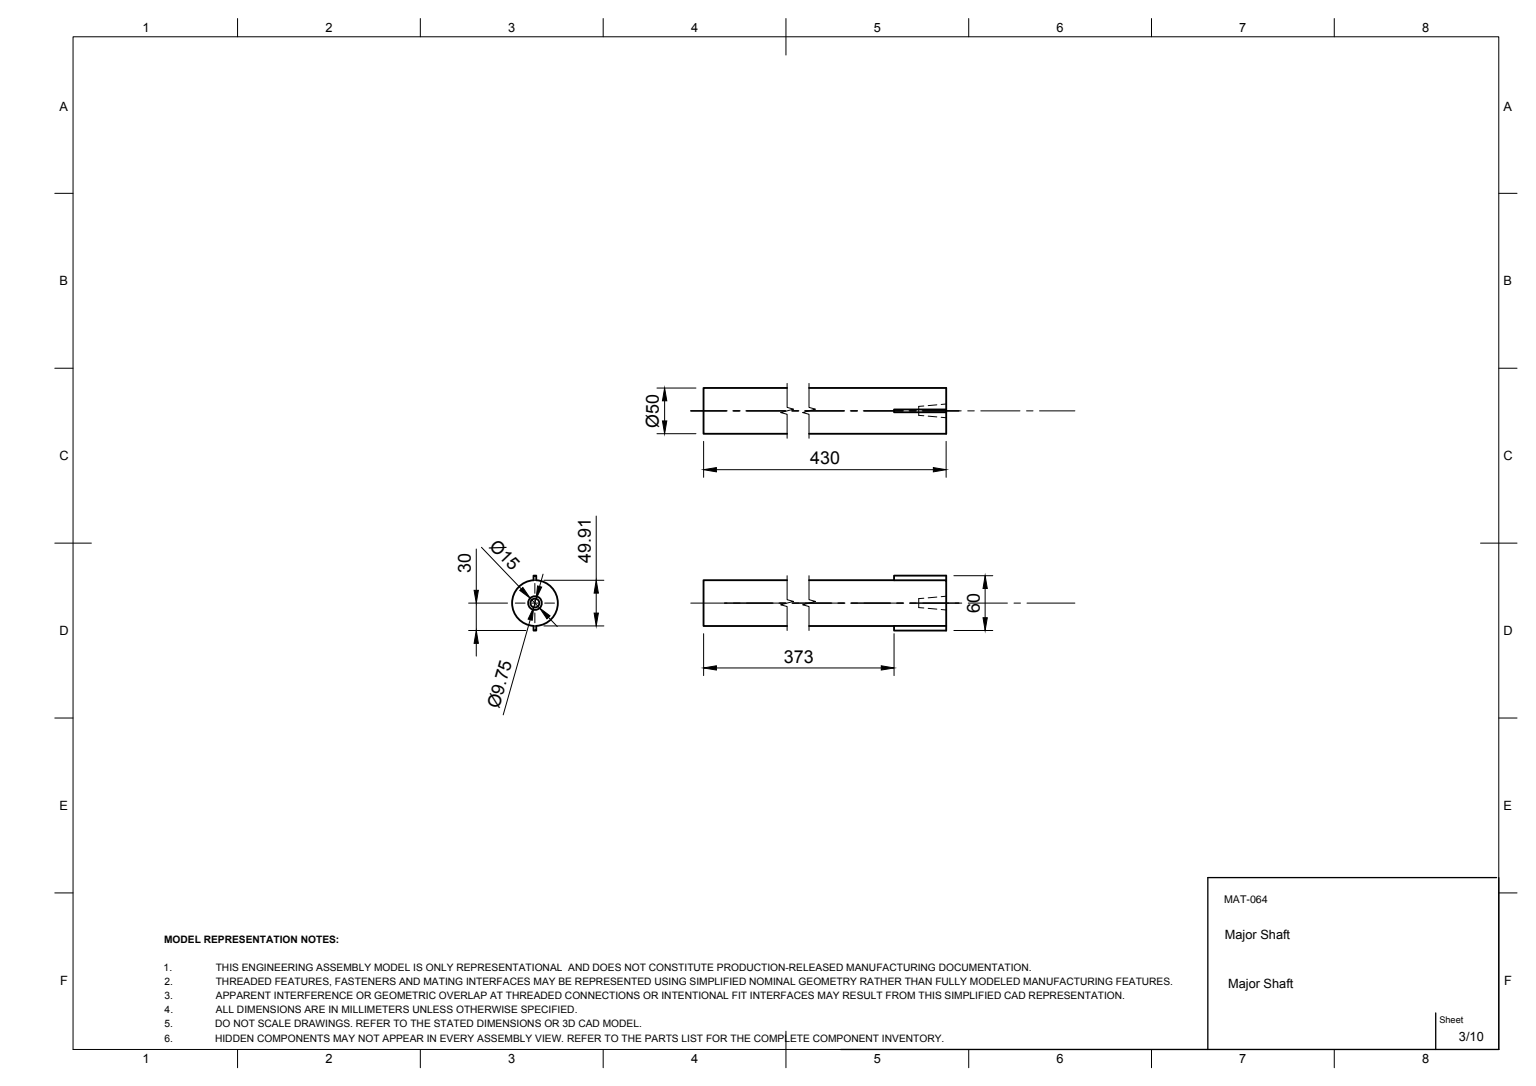
ISO-10303-21;
HEADER;
/* Generated by software containing ST-Developer
 * from STEP Tools, Inc. (www.steptools.com) 
 */

FILE_DESCRIPTION(
/* description */ (''),
/* implementation_level */ '2;1');

FILE_NAME(
/* name */ 
'Major Shaft.step',
/* time_stamp */ '2026-10-24T12:42:14-07:00',
/* author */ (''),
/* organization */ (''),
/* preprocessor_version */ 'ST-DEVELOPER v20.2',
/* originating_system */ 'Autodesk Translation Framework v15.15.0.0',
/* authorisation */ '');

FILE_SCHEMA (('AUTOMOTIVE_DESIGN { 1 0 10303 214 3 1 1 }'));
ENDSEC;

DATA;
#10=MECHANICAL_DESIGN_GEOMETRIC_PRESENTATION_REPRESENTATION('',(#68),#6789);
#15=CONICAL_SURFACE('',#4306,7.5,0.0872664625997165);
#56=SHAPE_REPRESENTATION_RELATIONSHIP('SRR','None',#6823,#62);
#62=ADVANCED_BREP_SHAPE_REPRESENTATION('',(#74),#6785);
#68=STYLED_ITEM('',(#6863),#74);
#74=MANIFOLD_SOLID_BREP('Major Shaft',#3963);
#160=CYLINDRICAL_SURFACE('',#4288,25.);
#219=FACE_BOUND('',#797,.T.);
#322=CIRCLE('',#4289,25.);
#323=CIRCLE('',#4290,25.);
#324=CIRCLE('',#4291,25.);
#325=CIRCLE('',#4292,25.);
#326=CIRCLE('',#4293,25.);
#327=CIRCLE('',#4294,25.);
#328=CIRCLE('',#4296,7.5);
#329=CIRCLE('',#4307,4.87534009422228);
#544=FACE_OUTER_BOUND('',#795,.T.);
#545=FACE_OUTER_BOUND('',#796,.T.);
#546=FACE_OUTER_BOUND('',#798,.T.);
#547=FACE_OUTER_BOUND('',#799,.T.);
#548=FACE_OUTER_BOUND('',#800,.T.);
#549=FACE_OUTER_BOUND('',#801,.T.);
#550=FACE_OUTER_BOUND('',#802,.T.);
#551=FACE_OUTER_BOUND('',#803,.T.);
#552=FACE_OUTER_BOUND('',#804,.T.);
#553=FACE_OUTER_BOUND('',#805,.T.);
#554=FACE_OUTER_BOUND('',#806,.T.);
#555=FACE_OUTER_BOUND('',#807,.T.);
#556=FACE_OUTER_BOUND('',#808,.T.);
#795=EDGE_LOOP('',(#3345,#3346,#3347,#3348,#3349,#3350,#3351,#3352,#3353,
#3354,#3355,#3356));
#796=EDGE_LOOP('',(#3357,#3358,#3359,#3360,#3361,#3362,#3363,#3364));
#797=EDGE_LOOP('',(#3365));
#798=EDGE_LOOP('',(#3366));
#799=EDGE_LOOP('',(#3367,#3368,#3369,#3370,#3371));
#800=EDGE_LOOP('',(#3372,#3373,#3374,#3375));
#801=EDGE_LOOP('',(#3376,#3377,#3378,#3379));
#802=EDGE_LOOP('',(#3380,#3381,#3382,#3383));
#803=EDGE_LOOP('',(#3384,#3385,#3386,#3387));
#804=EDGE_LOOP('',(#3388,#3389,#3390,#3391));
#805=EDGE_LOOP('',(#3392,#3393,#3394,#3395));
#806=EDGE_LOOP('',(#3396,#3397,#3398,#3399));
#807=EDGE_LOOP('',(#3400,#3401,#3402,#3403));
#808=EDGE_LOOP('',(#3404));
#1195=LINE('',#6434,#1573);
#1196=LINE('',#6438,#1574);
#1197=LINE('',#6442,#1575);
#1198=LINE('',#6446,#1576);
#1199=LINE('',#6450,#1577);
#1200=LINE('',#6454,#1578);
#1201=LINE('',#6456,#1579);
#1202=LINE('',#6457,#1580);
#1203=LINE('',#6459,#1581);
#1204=LINE('',#6461,#1582);
#1205=LINE('',#6462,#1583);
#1206=LINE('',#6469,#1584);
#1207=LINE('',#6470,#1585);
#1208=LINE('',#6471,#1586);
#1209=LINE('',#6473,#1587);
#1210=LINE('',#6475,#1588);
#1211=LINE('',#6479,#1589);
#1212=LINE('',#6481,#1590);
#1213=LINE('',#6482,#1591);
#1214=LINE('',#6484,#1592);
#1215=LINE('',#6486,#1593);
#1216=LINE('',#6491,#1594);
#1573=VECTOR('',#5254,25.);
#1574=VECTOR('',#5257,57.0000000000001);
#1575=VECTOR('',#5260,57.0000000000001);
#1576=VECTOR('',#5263,57.0000000000001);
#1577=VECTOR('',#5266,57.0000000000001);
#1578=VECTOR('',#5271,5.04504057306444);
#1579=VECTOR('',#5272,3.);
#1580=VECTOR('',#5273,5.04504057306444);
#1581=VECTOR('',#5274,5.04504057306444);
#1582=VECTOR('',#5275,3.);
#1583=VECTOR('',#5276,5.04504057306444);
#1584=VECTOR('',#5283,3.);
#1585=VECTOR('',#5284,5.04504057306444);
#1586=VECTOR('',#5285,5.04504057306444);
#1587=VECTOR('',#5288,57.0000000000001);
#1588=VECTOR('',#5291,57.0000000000001);
#1589=VECTOR('',#5296,5.04504057306444);
#1590=VECTOR('',#5297,3.);
#1591=VECTOR('',#5298,5.04504057306444);
#1592=VECTOR('',#5301,57.0000000000001);
#1593=VECTOR('',#5304,57.0000000000001);
#1594=VECTOR('',#5311,7.5);
#1901=VERTEX_POINT('',#6431);
#1902=VERTEX_POINT('',#6433);
#1903=VERTEX_POINT('',#6435);
#1904=VERTEX_POINT('',#6437);
#1905=VERTEX_POINT('',#6439);
#1906=VERTEX_POINT('',#6441);
#1907=VERTEX_POINT('',#6443);
#1908=VERTEX_POINT('',#6445);
#1909=VERTEX_POINT('',#6447);
#1910=VERTEX_POINT('',#6449);
#1911=VERTEX_POINT('',#6453);
#1912=VERTEX_POINT('',#6455);
#1913=VERTEX_POINT('',#6458);
#1914=VERTEX_POINT('',#6460);
#1915=VERTEX_POINT('',#6463);
#1916=VERTEX_POINT('',#6467);
#1917=VERTEX_POINT('',#6468);
#1918=VERTEX_POINT('',#6478);
#1919=VERTEX_POINT('',#6480);
#1920=VERTEX_POINT('',#6489);
#2393=EDGE_CURVE('',#1901,#1901,#322,.T.);
#2394=EDGE_CURVE('',#1901,#1902,#1195,.T.);
#2395=EDGE_CURVE('',#1902,#1903,#323,.T.);
#2396=EDGE_CURVE('',#1903,#1904,#1196,.T.);
#2397=EDGE_CURVE('',#1904,#1905,#324,.T.);
#2398=EDGE_CURVE('',#1906,#1905,#1197,.T.);
#2399=EDGE_CURVE('',#1906,#1907,#325,.T.);
#2400=EDGE_CURVE('',#1907,#1908,#1198,.T.);
#2401=EDGE_CURVE('',#1908,#1909,#326,.T.);
#2402=EDGE_CURVE('',#1910,#1909,#1199,.T.);
#2403=EDGE_CURVE('',#1910,#1902,#327,.T.);
#2404=EDGE_CURVE('',#1908,#1911,#1200,.T.);
#2405=EDGE_CURVE('',#1911,#1912,#1201,.T.);
#2406=EDGE_CURVE('',#1912,#1905,#1202,.T.);
#2407=EDGE_CURVE('',#1904,#1913,#1203,.T.);
#2408=EDGE_CURVE('',#1913,#1914,#1204,.T.);
#2409=EDGE_CURVE('',#1914,#1909,#1205,.T.);
#2410=EDGE_CURVE('',#1915,#1915,#328,.T.);
#2411=EDGE_CURVE('',#1916,#1917,#1206,.T.);
#2412=EDGE_CURVE('',#1903,#1916,#1207,.T.);
#2413=EDGE_CURVE('',#1917,#1910,#1208,.T.);
#2414=EDGE_CURVE('',#1917,#1914,#1209,.T.);
#2415=EDGE_CURVE('',#1916,#1913,#1210,.T.);
#2416=EDGE_CURVE('',#1918,#1906,#1211,.T.);
#2417=EDGE_CURVE('',#1919,#1918,#1212,.T.);
#2418=EDGE_CURVE('',#1907,#1919,#1213,.T.);
#2419=EDGE_CURVE('',#1919,#1911,#1214,.T.);
#2420=EDGE_CURVE('',#1918,#1912,#1215,.T.);
#2421=EDGE_CURVE('',#1920,#1920,#329,.T.);
#2422=EDGE_CURVE('',#1920,#1915,#1216,.T.);
#3345=ORIENTED_EDGE('',*,*,#2393,.F.);
#3346=ORIENTED_EDGE('',*,*,#2394,.T.);
#3347=ORIENTED_EDGE('',*,*,#2395,.T.);
#3348=ORIENTED_EDGE('',*,*,#2396,.T.);
#3349=ORIENTED_EDGE('',*,*,#2397,.T.);
#3350=ORIENTED_EDGE('',*,*,#2398,.F.);
#3351=ORIENTED_EDGE('',*,*,#2399,.T.);
#3352=ORIENTED_EDGE('',*,*,#2400,.T.);
#3353=ORIENTED_EDGE('',*,*,#2401,.T.);
#3354=ORIENTED_EDGE('',*,*,#2402,.F.);
#3355=ORIENTED_EDGE('',*,*,#2403,.T.);
#3356=ORIENTED_EDGE('',*,*,#2394,.F.);
#3357=ORIENTED_EDGE('',*,*,#2401,.F.);
#3358=ORIENTED_EDGE('',*,*,#2404,.T.);
#3359=ORIENTED_EDGE('',*,*,#2405,.T.);
#3360=ORIENTED_EDGE('',*,*,#2406,.T.);
#3361=ORIENTED_EDGE('',*,*,#2397,.F.);
#3362=ORIENTED_EDGE('',*,*,#2407,.T.);
#3363=ORIENTED_EDGE('',*,*,#2408,.T.);
#3364=ORIENTED_EDGE('',*,*,#2409,.T.);
#3365=ORIENTED_EDGE('',*,*,#2410,.F.);
#3366=ORIENTED_EDGE('',*,*,#2393,.T.);
#3367=ORIENTED_EDGE('',*,*,#2411,.F.);
#3368=ORIENTED_EDGE('',*,*,#2412,.F.);
#3369=ORIENTED_EDGE('',*,*,#2395,.F.);
#3370=ORIENTED_EDGE('',*,*,#2403,.F.);
#3371=ORIENTED_EDGE('',*,*,#2413,.F.);
#3372=ORIENTED_EDGE('',*,*,#2414,.F.);
#3373=ORIENTED_EDGE('',*,*,#2413,.T.);
#3374=ORIENTED_EDGE('',*,*,#2402,.T.);
#3375=ORIENTED_EDGE('',*,*,#2409,.F.);
#3376=ORIENTED_EDGE('',*,*,#2396,.F.);
#3377=ORIENTED_EDGE('',*,*,#2412,.T.);
#3378=ORIENTED_EDGE('',*,*,#2415,.T.);
#3379=ORIENTED_EDGE('',*,*,#2407,.F.);
#3380=ORIENTED_EDGE('',*,*,#2415,.F.);
#3381=ORIENTED_EDGE('',*,*,#2411,.T.);
#3382=ORIENTED_EDGE('',*,*,#2414,.T.);
#3383=ORIENTED_EDGE('',*,*,#2408,.F.);
#3384=ORIENTED_EDGE('',*,*,#2416,.F.);
#3385=ORIENTED_EDGE('',*,*,#2417,.F.);
#3386=ORIENTED_EDGE('',*,*,#2418,.F.);
#3387=ORIENTED_EDGE('',*,*,#2399,.F.);
#3388=ORIENTED_EDGE('',*,*,#2400,.F.);
#3389=ORIENTED_EDGE('',*,*,#2418,.T.);
#3390=ORIENTED_EDGE('',*,*,#2419,.T.);
#3391=ORIENTED_EDGE('',*,*,#2404,.F.);
#3392=ORIENTED_EDGE('',*,*,#2419,.F.);
#3393=ORIENTED_EDGE('',*,*,#2417,.T.);
#3394=ORIENTED_EDGE('',*,*,#2420,.T.);
#3395=ORIENTED_EDGE('',*,*,#2405,.F.);
#3396=ORIENTED_EDGE('',*,*,#2420,.F.);
#3397=ORIENTED_EDGE('',*,*,#2416,.T.);
#3398=ORIENTED_EDGE('',*,*,#2398,.T.);
#3399=ORIENTED_EDGE('',*,*,#2406,.F.);
#3400=ORIENTED_EDGE('',*,*,#2421,.F.);
#3401=ORIENTED_EDGE('',*,*,#2422,.T.);
#3402=ORIENTED_EDGE('',*,*,#2410,.T.);
#3403=ORIENTED_EDGE('',*,*,#2422,.F.);
#3404=ORIENTED_EDGE('',*,*,#2421,.T.);
#3715=PLANE('',#4295);
#3716=PLANE('',#4297);
#3717=PLANE('',#4298);
#3718=PLANE('',#4299);
#3719=PLANE('',#4300);
#3720=PLANE('',#4301);
#3721=PLANE('',#4302);
#3722=PLANE('',#4303);
#3723=PLANE('',#4304);
#3724=PLANE('',#4305);
#3725=PLANE('',#4308);
#3894=ADVANCED_FACE('',(#544),#160,.T.);
#3895=ADVANCED_FACE('',(#545,#219),#3715,.F.);
#3896=ADVANCED_FACE('',(#546),#3716,.T.);
#3897=ADVANCED_FACE('',(#547),#3717,.T.);
#3898=ADVANCED_FACE('',(#548),#3718,.T.);
#3899=ADVANCED_FACE('',(#549),#3719,.T.);
#3900=ADVANCED_FACE('',(#550),#3720,.T.);
#3901=ADVANCED_FACE('',(#551),#3721,.T.);
#3902=ADVANCED_FACE('',(#552),#3722,.T.);
#3903=ADVANCED_FACE('',(#553),#3723,.T.);
#3904=ADVANCED_FACE('',(#554),#3724,.T.);
#3905=ADVANCED_FACE('',(#555),#15,.F.);
#3906=ADVANCED_FACE('',(#556),#3725,.T.);
#3963=CLOSED_SHELL('',(#3894,#3895,#3896,#3897,#3898,#3899,#3900,#3901,
#3902,#3903,#3904,#3905,#3906));
#4287=AXIS2_PLACEMENT_3D('',#6429,#5248,#5249);
#4288=AXIS2_PLACEMENT_3D('',#6430,#5250,#5251);
#4289=AXIS2_PLACEMENT_3D('',#6432,#5252,#5253);
#4290=AXIS2_PLACEMENT_3D('',#6436,#5255,#5256);
#4291=AXIS2_PLACEMENT_3D('',#6440,#5258,#5259);
#4292=AXIS2_PLACEMENT_3D('',#6444,#5261,#5262);
#4293=AXIS2_PLACEMENT_3D('',#6448,#5264,#5265);
#4294=AXIS2_PLACEMENT_3D('',#6451,#5267,#5268);
#4295=AXIS2_PLACEMENT_3D('',#6452,#5269,#5270);
#4296=AXIS2_PLACEMENT_3D('',#6464,#5277,#5278);
#4297=AXIS2_PLACEMENT_3D('',#6465,#5279,#5280);
#4298=AXIS2_PLACEMENT_3D('',#6466,#5281,#5282);
#4299=AXIS2_PLACEMENT_3D('',#6472,#5286,#5287);
#4300=AXIS2_PLACEMENT_3D('',#6474,#5289,#5290);
#4301=AXIS2_PLACEMENT_3D('',#6476,#5292,#5293);
#4302=AXIS2_PLACEMENT_3D('',#6477,#5294,#5295);
#4303=AXIS2_PLACEMENT_3D('',#6483,#5299,#5300);
#4304=AXIS2_PLACEMENT_3D('',#6485,#5302,#5303);
#4305=AXIS2_PLACEMENT_3D('',#6487,#5305,#5306);
#4306=AXIS2_PLACEMENT_3D('',#6488,#5307,#5308);
#4307=AXIS2_PLACEMENT_3D('',#6490,#5309,#5310);
#4308=AXIS2_PLACEMENT_3D('',#6492,#5312,#5313);
#5248=DIRECTION('axis',(0.,0.,1.));
#5249=DIRECTION('refdir',(1.,0.,0.));
#5250=DIRECTION('center_axis',(0.,-1.,0.));
#5251=DIRECTION('ref_axis',(0.,0.,-1.));
#5252=DIRECTION('center_axis',(0.,-1.,0.));
#5253=DIRECTION('ref_axis',(0.,0.,-1.));
#5254=DIRECTION('',(0.,1.,0.));
#5255=DIRECTION('center_axis',(0.,-1.,0.));
#5256=DIRECTION('ref_axis',(0.,0.,-1.));
#5257=DIRECTION('',(0.,1.,0.));
#5258=DIRECTION('center_axis',(0.,-1.,0.));
#5259=DIRECTION('ref_axis',(0.,0.,-1.));
#5260=DIRECTION('',(0.,1.,0.));
#5261=DIRECTION('center_axis',(0.,-1.,0.));
#5262=DIRECTION('ref_axis',(0.,0.,-1.));
#5263=DIRECTION('',(0.,1.,0.));
#5264=DIRECTION('center_axis',(0.,-1.,0.));
#5265=DIRECTION('ref_axis',(0.,0.,-1.));
#5266=DIRECTION('',(0.,1.,0.));
#5267=DIRECTION('center_axis',(0.,-1.,0.));
#5268=DIRECTION('ref_axis',(0.,0.,-1.));
#5269=DIRECTION('center_axis',(0.,-1.,0.));
#5270=DIRECTION('ref_axis',(0.,0.,-1.));
#5271=DIRECTION('',(2.75077823593892E-16,0.,-1.));
#5272=DIRECTION('',(-1.,0.,0.));
#5273=DIRECTION('',(4.95140082469005E-16,0.,1.));
#5274=DIRECTION('',(-4.95140082469005E-16,0.,1.));
#5275=DIRECTION('',(1.,0.,0.));
#5276=DIRECTION('',(-2.75077823593892E-16,0.,-1.));
#5277=DIRECTION('center_axis',(0.,1.,0.));
#5278=DIRECTION('ref_axis',(0.,0.,1.));
#5279=DIRECTION('center_axis',(0.,-1.,0.));
#5280=DIRECTION('ref_axis',(0.,0.,-1.));
#5281=DIRECTION('center_axis',(0.,-1.,0.));
#5282=DIRECTION('ref_axis',(0.,0.,-1.));
#5283=DIRECTION('',(1.,0.,0.));
#5284=DIRECTION('',(-4.95140082469005E-16,0.,1.));
#5285=DIRECTION('',(-2.75077823593892E-16,0.,-1.));
#5286=DIRECTION('center_axis',(1.,0.,-3.00866369555819E-16));
#5287=DIRECTION('ref_axis',(-3.00866369555819E-16,0.,-1.));
#5288=DIRECTION('',(0.,1.,0.));
#5289=DIRECTION('center_axis',(-1.,0.,-4.72790009302002E-16));
#5290=DIRECTION('ref_axis',(-4.72790009302002E-16,0.,1.));
#5291=DIRECTION('',(0.,1.,0.));
#5292=DIRECTION('center_axis',(0.,0.,1.));
#5293=DIRECTION('ref_axis',(1.,0.,0.));
#5294=DIRECTION('center_axis',(0.,-1.,0.));
#5295=DIRECTION('ref_axis',(0.,0.,-1.));
#5296=DIRECTION('',(4.95140082469005E-16,0.,1.));
#5297=DIRECTION('',(-1.,0.,0.));
#5298=DIRECTION('',(2.75077823593892E-16,0.,-1.));
#5299=DIRECTION('center_axis',(1.,0.,3.00866369555819E-16));
#5300=DIRECTION('ref_axis',(3.00866369555819E-16,0.,-1.));
#5301=DIRECTION('',(0.,1.,0.));
#5302=DIRECTION('center_axis',(0.,0.,-1.));
#5303=DIRECTION('ref_axis',(-1.,0.,0.));
#5304=DIRECTION('',(0.,1.,0.));
#5305=DIRECTION('center_axis',(-1.,0.,4.72790009302002E-16));
#5306=DIRECTION('ref_axis',(4.72790009302002E-16,0.,1.));
#5307=DIRECTION('center_axis',(0.,1.,0.));
#5308=DIRECTION('ref_axis',(0.,0.,1.));
#5309=DIRECTION('center_axis',(0.,1.,0.));
#5310=DIRECTION('ref_axis',(0.,0.,1.));
#5311=DIRECTION('',(-1.0673500138323E-17,0.996194698091745,-0.0871557427476582));
#5312=DIRECTION('center_axis',(0.,1.,0.));
#5313=DIRECTION('ref_axis',(0.,0.,1.));
#6429=CARTESIAN_POINT('',(0.,0.,0.));
#6430=CARTESIAN_POINT('Origin',(0.,42.0000000000001,0.));
#6431=CARTESIAN_POINT('',(-3.06161699786838E-15,-388.,25.));
#6432=CARTESIAN_POINT('Origin',(0.,-388.,0.));
#6433=CARTESIAN_POINT('',(-3.06161699786838E-15,-15.,25.));
#6434=CARTESIAN_POINT('',(-3.06161699786838E-15,42.0000000000001,25.));
#6435=CARTESIAN_POINT('',(-1.5,-15.,24.9549594269356));
#6436=CARTESIAN_POINT('Origin',(0.,-15.,0.));
#6437=CARTESIAN_POINT('',(-1.5,42.0000000000001,24.9549594269356));
#6438=CARTESIAN_POINT('',(-1.5,-15.,24.9549594269356));
#6439=CARTESIAN_POINT('',(-1.5,42.0000000000001,-24.9549594269356));
#6440=CARTESIAN_POINT('Origin',(0.,42.0000000000001,0.));
#6441=CARTESIAN_POINT('',(-1.5,-15.,-24.9549594269356));
#6442=CARTESIAN_POINT('',(-1.49999999999999,-15.,-24.9549594269356));
#6443=CARTESIAN_POINT('',(1.5,-15.,-24.9549594269356));
#6444=CARTESIAN_POINT('Origin',(0.,-15.,0.));
#6445=CARTESIAN_POINT('',(1.5,42.0000000000001,-24.9549594269356));
#6446=CARTESIAN_POINT('',(1.5,-15.,-24.9549594269356));
#6447=CARTESIAN_POINT('',(1.5,42.0000000000001,24.9549594269356));
#6448=CARTESIAN_POINT('Origin',(0.,42.0000000000001,0.));
#6449=CARTESIAN_POINT('',(1.5,-15.,24.9549594269356));
#6450=CARTESIAN_POINT('',(1.5,-15.,24.9549594269356));
#6451=CARTESIAN_POINT('Origin',(0.,-15.,0.));
#6452=CARTESIAN_POINT('Origin',(0.,42.0000000000001,0.));
#6453=CARTESIAN_POINT('',(1.5,42.0000000000001,-30.));
#6454=CARTESIAN_POINT('',(1.5,42.0000000000001,-24.9549594269356));
#6455=CARTESIAN_POINT('',(-1.5,42.0000000000001,-30.));
#6456=CARTESIAN_POINT('',(1.5,42.0000000000001,-30.));
#6457=CARTESIAN_POINT('',(-1.5,42.0000000000001,-30.));
#6458=CARTESIAN_POINT('',(-1.5,42.0000000000001,30.));
#6459=CARTESIAN_POINT('',(-1.5,42.0000000000001,24.9549594269356));
#6460=CARTESIAN_POINT('',(1.5,42.0000000000001,30.));
#6461=CARTESIAN_POINT('',(-1.5,42.0000000000001,30.));
#6462=CARTESIAN_POINT('',(1.5,42.0000000000001,30.));
#6463=CARTESIAN_POINT('',(-9.18485099360515E-16,42.0000000000001,-7.5));
#6464=CARTESIAN_POINT('Origin',(0.,42.0000000000001,0.));
#6465=CARTESIAN_POINT('Origin',(0.,-388.,0.));
#6466=CARTESIAN_POINT('Origin',(0.,-15.,0.));
#6467=CARTESIAN_POINT('',(-1.5,-15.,30.));
#6468=CARTESIAN_POINT('',(1.5,-15.,30.));
#6469=CARTESIAN_POINT('',(-1.5,-15.,30.));
#6470=CARTESIAN_POINT('',(-1.5,-15.,24.9549594269356));
#6471=CARTESIAN_POINT('',(1.5,-15.,30.));
#6472=CARTESIAN_POINT('Origin',(1.5,-20.8696196115137,30.));
#6473=CARTESIAN_POINT('',(1.5,-15.,30.));
#6474=CARTESIAN_POINT('Origin',(-1.5,-20.8696196115137,30.));
#6475=CARTESIAN_POINT('',(-1.5,-15.,30.));
#6476=CARTESIAN_POINT('Origin',(-1.5,-20.8696196115137,30.));
#6477=CARTESIAN_POINT('Origin',(0.,-15.,0.));
#6478=CARTESIAN_POINT('',(-1.5,-15.,-30.));
#6479=CARTESIAN_POINT('',(-1.5,-15.,-30.));
#6480=CARTESIAN_POINT('',(1.5,-15.,-30.));
#6481=CARTESIAN_POINT('',(1.5,-15.,-30.));
#6482=CARTESIAN_POINT('',(1.5,-15.,-24.9549594269356));
#6483=CARTESIAN_POINT('Origin',(1.5,-20.8696196115137,-30.));
#6484=CARTESIAN_POINT('',(1.5,-15.,-30.));
#6485=CARTESIAN_POINT('Origin',(-1.5,-20.8696196115137,-30.));
#6486=CARTESIAN_POINT('',(-1.5,-15.,-30.));
#6487=CARTESIAN_POINT('Origin',(-1.5,-20.8696196115137,-30.));
#6488=CARTESIAN_POINT('Origin',(0.,42.0000000000001,0.));
#6489=CARTESIAN_POINT('',(-5.97056964114407E-16,12.0000000000001,-4.87534009422228));
#6490=CARTESIAN_POINT('Origin',(0.,12.0000000000001,0.));
#6491=CARTESIAN_POINT('',(-9.18485099360515E-16,42.0000000000001,-7.5));
#6492=CARTESIAN_POINT('Origin',(0.,12.0000000000001,0.));
#6776=UNCERTAINTY_MEASURE_WITH_UNIT(LENGTH_MEASURE(0.01),#6790,
'DISTANCE_ACCURACY_VALUE',
'Maximum model space distance between geometric entities at asserted c
onnectivities');
#6780=UNCERTAINTY_MEASURE_WITH_UNIT(LENGTH_MEASURE(0.01),#6790,
'DISTANCE_ACCURACY_VALUE',
'Maximum model space distance between geometric entities at asserted c
onnectivities');
#6785=(
GEOMETRIC_REPRESENTATION_CONTEXT(3)
GLOBAL_UNCERTAINTY_ASSIGNED_CONTEXT((#6776))
GLOBAL_UNIT_ASSIGNED_CONTEXT((#6790,#6792,#6793))
REPRESENTATION_CONTEXT('','3D')
);
#6789=(
GEOMETRIC_REPRESENTATION_CONTEXT(3)
GLOBAL_UNCERTAINTY_ASSIGNED_CONTEXT((#6780))
GLOBAL_UNIT_ASSIGNED_CONTEXT((#6790,#6792,#6793))
REPRESENTATION_CONTEXT('','3D')
);
#6790=(
LENGTH_UNIT()
NAMED_UNIT(*)
SI_UNIT(.MILLI.,.METRE.)
);
#6792=(
NAMED_UNIT(*)
PLANE_ANGLE_UNIT()
SI_UNIT($,.RADIAN.)
);
#6793=(
NAMED_UNIT(*)
SI_UNIT($,.STERADIAN.)
SOLID_ANGLE_UNIT()
);
#6798=SHAPE_DEFINITION_REPRESENTATION(#6809,#6823);
#6809=PRODUCT_DEFINITION_SHAPE('',$,#6832);
#6823=SHAPE_REPRESENTATION('',(#4287),#6785);
#6827=PRODUCT_DEFINITION_CONTEXT('part definition',#6853,'design');
#6832=PRODUCT_DEFINITION('Major Shaft','Major Shaft',#6840,#6827);
#6840=PRODUCT_DEFINITION_FORMATION('',$,#6859);
#6853=APPLICATION_CONTEXT(
'Core Data for Automotive Mechanical Design Process');
#6854=PRODUCT_CONTEXT('part definition',#6853,'mechanical');
#6859=PRODUCT('Major Shaft','Major Shaft',$,(#6854));
#6863=PRESENTATION_STYLE_ASSIGNMENT((#6865));
#6865=SURFACE_STYLE_USAGE(.BOTH.,#6867);
#6867=SURFACE_SIDE_STYLE('',(#6869));
#6869=SURFACE_STYLE_FILL_AREA(#6871);
#6871=FILL_AREA_STYLE('Steel - Satin',(#6873));
#6873=FILL_AREA_STYLE_COLOUR('Steel - Satin',#6875);
#6875=COLOUR_RGB('Steel - Satin',0.627450980392157,0.627450980392157,0.627450980392157);
ENDSEC;
END-ISO-10303-21;
